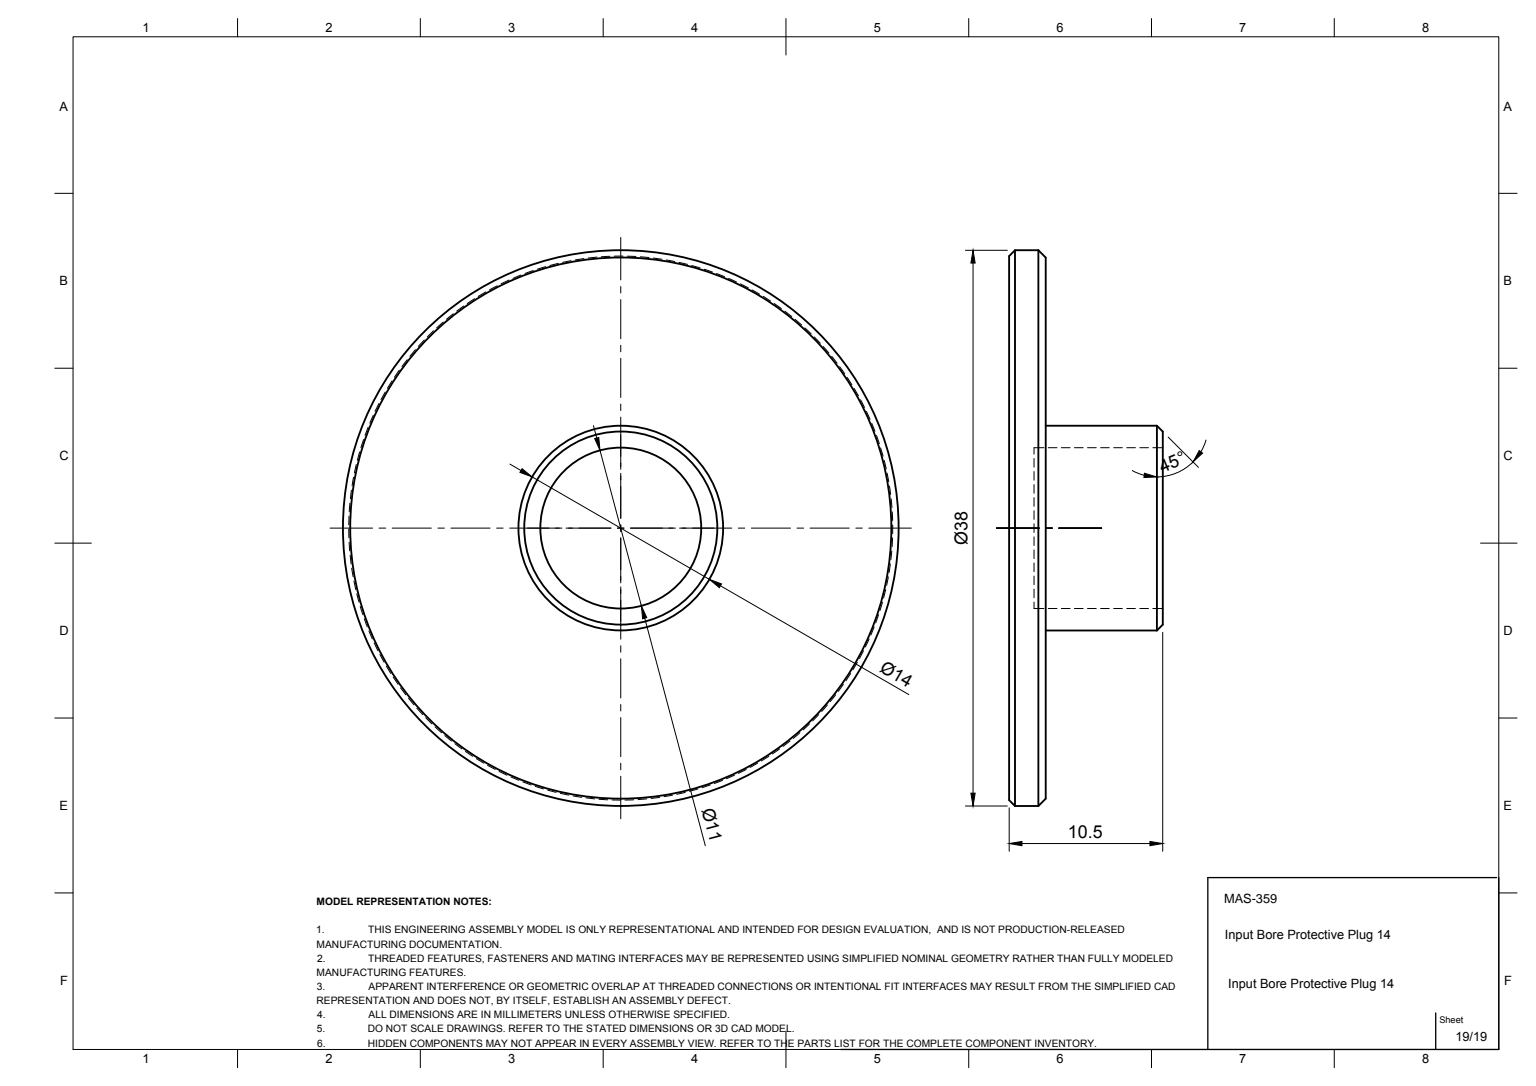
ISO-10303-21;
HEADER;
/* Generated by software containing ST-Developer
 * from STEP Tools, Inc. (www.steptools.com) 
 */

FILE_DESCRIPTION(
/* description */ (''),
/* implementation_level */ '2;1');

FILE_NAME(
/* name */ 'Input Bore Protective Plug 14.step',
/* time_stamp */ '2026-10-15T14:25:16-07:00',
/* author */ (''),
/* organization */ (''),
/* preprocessor_version */ 'ST-DEVELOPER v20.2',
/* originating_system */ 'Autodesk Translation Framework v15.15.0.0',
/* authorisation */ '');

FILE_SCHEMA (('AUTOMOTIVE_DESIGN { 1 0 10303 214 3 1 1 }'));
ENDSEC;

DATA;
#10=MECHANICAL_DESIGN_GEOMETRIC_PRESENTATION_REPRESENTATION('',(#333),#86429);
#297=SHAPE_REPRESENTATION_RELATIONSHIP('SRR','None',#86512,#315);
#315=ADVANCED_BREP_SHAPE_REPRESENTATION('',(#351),#86421);
#333=STYLED_ITEM('',(#86611),#351);
#351=MANIFOLD_SOLID_BREP('Body1',#15623);
#1318=CONICAL_SURFACE('',#16971,0.68,0.785398163397448);
#1319=CONICAL_SURFACE('',#16977,1.875,0.785398163397447);
#1320=CONICAL_SURFACE('',#16981,1.88,0.785398163397446);
#1532=CYLINDRICAL_SURFACE('',#16966,0.55);
#1533=CYLINDRICAL_SURFACE('',#16973,0.7);
#1534=CYLINDRICAL_SURFACE('',#16979,1.9);
#1723=FACE_BOUND('',#4088,.T.);
#1724=FACE_BOUND('',#4092,.T.);
#2261=CIRCLE('',#16967,0.55);
#2262=CIRCLE('',#16968,0.55);
#2263=CIRCLE('',#16970,0.66);
#2264=CIRCLE('',#16972,0.7);
#2265=CIRCLE('',#16974,0.7);
#2266=CIRCLE('',#16976,1.85);
#2267=CIRCLE('',#16978,1.9);
#2268=CIRCLE('',#16980,1.9);
#2269=CIRCLE('',#16982,1.86);
#3093=FACE_OUTER_BOUND('',#4086,.T.);
#3094=FACE_OUTER_BOUND('',#4087,.T.);
#3095=FACE_OUTER_BOUND('',#4089,.T.);
#3096=FACE_OUTER_BOUND('',#4090,.T.);
#3097=FACE_OUTER_BOUND('',#4091,.T.);
#3098=FACE_OUTER_BOUND('',#4093,.T.);
#3099=FACE_OUTER_BOUND('',#4094,.T.);
#3100=FACE_OUTER_BOUND('',#4095,.T.);
#3101=FACE_OUTER_BOUND('',#4096,.T.);
#3102=FACE_OUTER_BOUND('',#4097,.T.);
#4086=EDGE_LOOP('',(#13529,#13530,#13531,#13532));
#4087=EDGE_LOOP('',(#13533));
#4088=EDGE_LOOP('',(#13534));
#4089=EDGE_LOOP('',(#13535,#13536,#13537,#13538));
#4090=EDGE_LOOP('',(#13539,#13540,#13541,#13542));
#4091=EDGE_LOOP('',(#13543));
#4092=EDGE_LOOP('',(#13544));
#4093=EDGE_LOOP('',(#13545,#13546,#13547,#13548));
#4094=EDGE_LOOP('',(#13549,#13550,#13551,#13552));
#4095=EDGE_LOOP('',(#13553,#13554,#13555,#13556));
#4096=EDGE_LOOP('',(#13557));
#4097=EDGE_LOOP('',(#13558));
#5012=LINE('',#66343,#5872);
#5013=LINE('',#66351,#5873);
#5014=LINE('',#66355,#5874);
#5015=LINE('',#66362,#5875);
#5016=LINE('',#66366,#5876);
#5017=LINE('',#66369,#5877);
#5872=VECTOR('',#20293,0.55);
#5873=VECTOR('',#20304,0.68);
#5874=VECTOR('',#20309,0.7);
#5875=VECTOR('',#20318,1.875);
#5876=VECTOR('',#20323,1.9);
#5877=VECTOR('',#20326,1.88);
#7209=VERTEX_POINT('',#66340);
#7210=VERTEX_POINT('',#66342);
#7211=VERTEX_POINT('',#66346);
#7212=VERTEX_POINT('',#66349);
#7213=VERTEX_POINT('',#66353);
#7214=VERTEX_POINT('',#66357);
#7215=VERTEX_POINT('',#66360);
#7216=VERTEX_POINT('',#66364);
#7217=VERTEX_POINT('',#66368);
#9386=EDGE_CURVE('',#7209,#7209,#2261,.T.);
#9387=EDGE_CURVE('',#7209,#7210,#5012,.T.);
#9388=EDGE_CURVE('',#7210,#7210,#2262,.T.);
#9389=EDGE_CURVE('',#7211,#7211,#2263,.T.);
#9390=EDGE_CURVE('',#7212,#7212,#2264,.T.);
#9391=EDGE_CURVE('',#7212,#7211,#5013,.T.);
#9392=EDGE_CURVE('',#7213,#7213,#2265,.T.);
#9393=EDGE_CURVE('',#7213,#7212,#5014,.T.);
#9394=EDGE_CURVE('',#7214,#7214,#2266,.T.);
#9395=EDGE_CURVE('',#7215,#7215,#2267,.T.);
#9396=EDGE_CURVE('',#7215,#7214,#5015,.T.);
#9397=EDGE_CURVE('',#7216,#7216,#2268,.T.);
#9398=EDGE_CURVE('',#7216,#7215,#5016,.T.);
#9399=EDGE_CURVE('',#7216,#7217,#5017,.T.);
#9400=EDGE_CURVE('',#7217,#7217,#2269,.T.);
#13529=ORIENTED_EDGE('',*,*,#9386,.F.);
#13530=ORIENTED_EDGE('',*,*,#9387,.T.);
#13531=ORIENTED_EDGE('',*,*,#9388,.T.);
#13532=ORIENTED_EDGE('',*,*,#9387,.F.);
#13533=ORIENTED_EDGE('',*,*,#9389,.F.);
#13534=ORIENTED_EDGE('',*,*,#9386,.T.);
#13535=ORIENTED_EDGE('',*,*,#9390,.F.);
#13536=ORIENTED_EDGE('',*,*,#9391,.T.);
#13537=ORIENTED_EDGE('',*,*,#9389,.T.);
#13538=ORIENTED_EDGE('',*,*,#9391,.F.);
#13539=ORIENTED_EDGE('',*,*,#9392,.F.);
#13540=ORIENTED_EDGE('',*,*,#9393,.T.);
#13541=ORIENTED_EDGE('',*,*,#9390,.T.);
#13542=ORIENTED_EDGE('',*,*,#9393,.F.);
#13543=ORIENTED_EDGE('',*,*,#9394,.F.);
#13544=ORIENTED_EDGE('',*,*,#9392,.T.);
#13545=ORIENTED_EDGE('',*,*,#9395,.F.);
#13546=ORIENTED_EDGE('',*,*,#9396,.T.);
#13547=ORIENTED_EDGE('',*,*,#9394,.T.);
#13548=ORIENTED_EDGE('',*,*,#9396,.F.);
#13549=ORIENTED_EDGE('',*,*,#9397,.F.);
#13550=ORIENTED_EDGE('',*,*,#9398,.T.);
#13551=ORIENTED_EDGE('',*,*,#9395,.T.);
#13552=ORIENTED_EDGE('',*,*,#9398,.F.);
#13553=ORIENTED_EDGE('',*,*,#9397,.T.);
#13554=ORIENTED_EDGE('',*,*,#9399,.T.);
#13555=ORIENTED_EDGE('',*,*,#9400,.F.);
#13556=ORIENTED_EDGE('',*,*,#9399,.F.);
#13557=ORIENTED_EDGE('',*,*,#9400,.T.);
#13558=ORIENTED_EDGE('',*,*,#9388,.F.);
#14688=PLANE('',#16969);
#14689=PLANE('',#16975);
#14690=PLANE('',#16983);
#14691=PLANE('',#16984);
#15449=ADVANCED_FACE('',(#3093),#1532,.F.);
#15450=ADVANCED_FACE('',(#3094,#1723),#14688,.T.);
#15451=ADVANCED_FACE('',(#3095),#1318,.T.);
#15452=ADVANCED_FACE('',(#3096),#1533,.T.);
#15453=ADVANCED_FACE('',(#3097,#1724),#14689,.T.);
#15454=ADVANCED_FACE('',(#3098),#1319,.T.);
#15455=ADVANCED_FACE('',(#3099),#1534,.T.);
#15456=ADVANCED_FACE('',(#3100),#1320,.T.);
#15457=ADVANCED_FACE('',(#3101),#14690,.T.);
#15458=ADVANCED_FACE('',(#3102),#14691,.T.);
#15623=CLOSED_SHELL('',(#15449,#15450,#15451,#15452,#15453,#15454,#15455,
#15456,#15457,#15458));
#16965=AXIS2_PLACEMENT_3D('',#66338,#20287,#20288);
#16966=AXIS2_PLACEMENT_3D('',#66339,#20289,#20290);
#16967=AXIS2_PLACEMENT_3D('',#66341,#20291,#20292);
#16968=AXIS2_PLACEMENT_3D('',#66344,#20294,#20295);
#16969=AXIS2_PLACEMENT_3D('',#66345,#20296,#20297);
#16970=AXIS2_PLACEMENT_3D('',#66347,#20298,#20299);
#16971=AXIS2_PLACEMENT_3D('',#66348,#20300,#20301);
#16972=AXIS2_PLACEMENT_3D('',#66350,#20302,#20303);
#16973=AXIS2_PLACEMENT_3D('',#66352,#20305,#20306);
#16974=AXIS2_PLACEMENT_3D('',#66354,#20307,#20308);
#16975=AXIS2_PLACEMENT_3D('',#66356,#20310,#20311);
#16976=AXIS2_PLACEMENT_3D('',#66358,#20312,#20313);
#16977=AXIS2_PLACEMENT_3D('',#66359,#20314,#20315);
#16978=AXIS2_PLACEMENT_3D('',#66361,#20316,#20317);
#16979=AXIS2_PLACEMENT_3D('',#66363,#20319,#20320);
#16980=AXIS2_PLACEMENT_3D('',#66365,#20321,#20322);
#16981=AXIS2_PLACEMENT_3D('',#66367,#20324,#20325);
#16982=AXIS2_PLACEMENT_3D('',#66370,#20327,#20328);
#16983=AXIS2_PLACEMENT_3D('',#66371,#20329,#20330);
#16984=AXIS2_PLACEMENT_3D('',#66372,#20331,#20332);
#20287=DIRECTION('axis',(0.,0.,1.));
#20288=DIRECTION('refdir',(1.,0.,0.));
#20289=DIRECTION('center_axis',(0.,0.,1.));
#20290=DIRECTION('ref_axis',(1.,0.,0.));
#20291=DIRECTION('center_axis',(0.,0.,1.));
#20292=DIRECTION('ref_axis',(1.,0.,0.));
#20293=DIRECTION('',(0.,0.,1.));
#20294=DIRECTION('center_axis',(0.,0.,1.));
#20295=DIRECTION('ref_axis',(1.,0.,0.));
#20296=DIRECTION('center_axis',(0.,0.,-1.));
#20297=DIRECTION('ref_axis',(-1.,0.,0.));
#20298=DIRECTION('center_axis',(0.,0.,1.));
#20299=DIRECTION('ref_axis',(1.,0.,0.));
#20300=DIRECTION('center_axis',(0.,0.,1.));
#20301=DIRECTION('ref_axis',(1.,0.,0.));
#20302=DIRECTION('center_axis',(0.,0.,1.));
#20303=DIRECTION('ref_axis',(1.,0.,0.));
#20304=DIRECTION('',(0.707106781186547,8.65956056235493E-17,-0.707106781186548));
#20305=DIRECTION('center_axis',(0.,0.,1.));
#20306=DIRECTION('ref_axis',(1.,0.,0.));
#20307=DIRECTION('center_axis',(0.,0.,1.));
#20308=DIRECTION('ref_axis',(1.,0.,0.));
#20309=DIRECTION('',(0.,0.,-1.));
#20310=DIRECTION('center_axis',(0.,0.,-1.));
#20311=DIRECTION('ref_axis',(-1.,0.,0.));
#20312=DIRECTION('center_axis',(0.,0.,1.));
#20313=DIRECTION('ref_axis',(1.,0.,0.));
#20314=DIRECTION('center_axis',(0.,0.,1.));
#20315=DIRECTION('ref_axis',(1.,0.,0.));
#20316=DIRECTION('center_axis',(0.,0.,1.));
#20317=DIRECTION('ref_axis',(1.,0.,0.));
#20318=DIRECTION('',(0.707106781186547,8.65956056235492E-17,-0.707106781186548));
#20319=DIRECTION('center_axis',(0.,0.,1.));
#20320=DIRECTION('ref_axis',(1.,0.,0.));
#20321=DIRECTION('center_axis',(0.,0.,1.));
#20322=DIRECTION('ref_axis',(1.,0.,0.));
#20323=DIRECTION('',(0.,0.,-1.));
#20324=DIRECTION('center_axis',(0.,0.,-1.));
#20325=DIRECTION('ref_axis',(1.,0.,0.));
#20326=DIRECTION('',(0.707106781186546,-8.65956056235491E-17,0.707106781186549));
#20327=DIRECTION('center_axis',(0.,0.,1.));
#20328=DIRECTION('ref_axis',(1.,0.,0.));
#20329=DIRECTION('center_axis',(0.,0.,1.));
#20330=DIRECTION('ref_axis',(1.,0.,0.));
#20331=DIRECTION('center_axis',(0.,0.,-1.));
#20332=DIRECTION('ref_axis',(-1.,0.,0.));
#66338=CARTESIAN_POINT('',(0.,0.,0.));
#66339=CARTESIAN_POINT('Origin',(0.,0.,-0.36));
#66340=CARTESIAN_POINT('',(-0.55,-6.73555739531044E-17,-0.8));
#66341=CARTESIAN_POINT('Origin',(0.,0.,-0.8));
#66342=CARTESIAN_POINT('',(-0.55,-6.73555739531044E-17,0.08));
#66343=CARTESIAN_POINT('',(-0.55,-6.73555739531044E-17,-0.36));
#66344=CARTESIAN_POINT('Origin',(0.,0.,0.08));
#66345=CARTESIAN_POINT('Origin',(0.66,0.,-0.8));
#66346=CARTESIAN_POINT('',(-0.66,-8.08266887437253E-17,-0.8));
#66347=CARTESIAN_POINT('Origin',(0.,0.,-0.8));
#66348=CARTESIAN_POINT('Origin',(0.,0.,-0.78));
#66349=CARTESIAN_POINT('',(-0.7,-8.57252759403147E-17,-0.76));
#66350=CARTESIAN_POINT('Origin',(0.,0.,-0.76));
#66351=CARTESIAN_POINT('',(-0.68,-8.327598234202E-17,-0.78));
#66352=CARTESIAN_POINT('Origin',(0.,0.,-0.38));
#66353=CARTESIAN_POINT('',(-0.7,-8.57252759403147E-17,0.));
#66354=CARTESIAN_POINT('Origin',(0.,0.,0.));
#66355=CARTESIAN_POINT('',(-0.7,-8.57252759403147E-17,-0.38));
#66356=CARTESIAN_POINT('Origin',(1.85,0.,0.));
#66357=CARTESIAN_POINT('',(-1.85,-2.2655965784226E-16,-2.42861286636753E-17));
#66358=CARTESIAN_POINT('Origin',(0.,0.,0.));
#66359=CARTESIAN_POINT('Origin',(0.,0.,0.025));
#66360=CARTESIAN_POINT('',(-1.9,-2.32682891837997E-16,0.05));
#66361=CARTESIAN_POINT('Origin',(0.,0.,0.05));
#66362=CARTESIAN_POINT('',(-1.875,-2.29621274840129E-16,0.025));
#66363=CARTESIAN_POINT('Origin',(0.,0.,0.13));
#66364=CARTESIAN_POINT('',(-1.9,-2.32682891837997E-16,0.21));
#66365=CARTESIAN_POINT('Origin',(0.,0.,0.21));
#66366=CARTESIAN_POINT('',(-1.9,-2.32682891837997E-16,0.13));
#66367=CARTESIAN_POINT('Origin',(0.,0.,0.23));
#66368=CARTESIAN_POINT('',(-1.86,-2.27784304641408E-16,0.25));
#66369=CARTESIAN_POINT('',(-1.88,2.30233598239702E-16,0.23));
#66370=CARTESIAN_POINT('Origin',(0.,0.,0.25));
#66371=CARTESIAN_POINT('Origin',(0.,0.,0.25));
#66372=CARTESIAN_POINT('Origin',(0.55,0.,0.08));
#86401=UNCERTAINTY_MEASURE_WITH_UNIT(LENGTH_MEASURE(0.001),#86430,
'DISTANCE_ACCURACY_VALUE',
'Maximum model space distance between geometric entities at asserted c
onnectivities');
#86409=UNCERTAINTY_MEASURE_WITH_UNIT(LENGTH_MEASURE(0.001),#86430,
'DISTANCE_ACCURACY_VALUE',
'Maximum model space distance between geometric entities at asserted c
onnectivities');
#86421=(
GEOMETRIC_REPRESENTATION_CONTEXT(3)
GLOBAL_UNCERTAINTY_ASSIGNED_CONTEXT((#86401))
GLOBAL_UNIT_ASSIGNED_CONTEXT((#86430,#86432,#86433))
REPRESENTATION_CONTEXT('','3D')
);
#86429=(
GEOMETRIC_REPRESENTATION_CONTEXT(3)
GLOBAL_UNCERTAINTY_ASSIGNED_CONTEXT((#86409))
GLOBAL_UNIT_ASSIGNED_CONTEXT((#86430,#86432,#86433))
REPRESENTATION_CONTEXT('','3D')
);
#86430=(
LENGTH_UNIT()
NAMED_UNIT(*)
SI_UNIT(.CENTI.,.METRE.)
);
#86432=(
NAMED_UNIT(*)
PLANE_ANGLE_UNIT()
SI_UNIT($,.RADIAN.)
);
#86433=(
NAMED_UNIT(*)
SI_UNIT($,.STERADIAN.)
SOLID_ANGLE_UNIT()
);
#86445=SHAPE_DEFINITION_REPRESENTATION(#86464,#86512);
#86464=PRODUCT_DEFINITION_SHAPE('',$,#86532);
#86512=SHAPE_REPRESENTATION('',(#16965),#86421);
#86520=PRODUCT_DEFINITION_CONTEXT('part definition',#86579,'design');
#86532=PRODUCT_DEFINITION('Input Bore Protective Plug 14',
'Input Bore Protective Plug 14',#86551,#86520);
#86551=PRODUCT_DEFINITION_FORMATION('',$,#86592);
#86579=APPLICATION_CONTEXT(
'Core Data for Automotive Mechanical Design Process');
#86580=PRODUCT_CONTEXT('part definition',#86579,'mechanical');
#86592=PRODUCT('Input Bore Protective Plug 14',
'Input Bore Protective Plug 14',$,(#86580));
#86611=PRESENTATION_STYLE_ASSIGNMENT((#86629));
#86629=SURFACE_STYLE_USAGE(.BOTH.,#86647);
#86647=SURFACE_SIDE_STYLE('',(#86665));
#86665=SURFACE_STYLE_FILL_AREA(#86683);
#86683=FILL_AREA_STYLE('Opaque(240,172,28)',(#86701));
#86701=FILL_AREA_STYLE_COLOUR('Opaque(240,172,28)',#86719);
#86719=COLOUR_RGB('Opaque(240,172,28)', 0.72549020, 0.75294118, 0.79215686);
ENDSEC;
END-ISO-10303-21;
